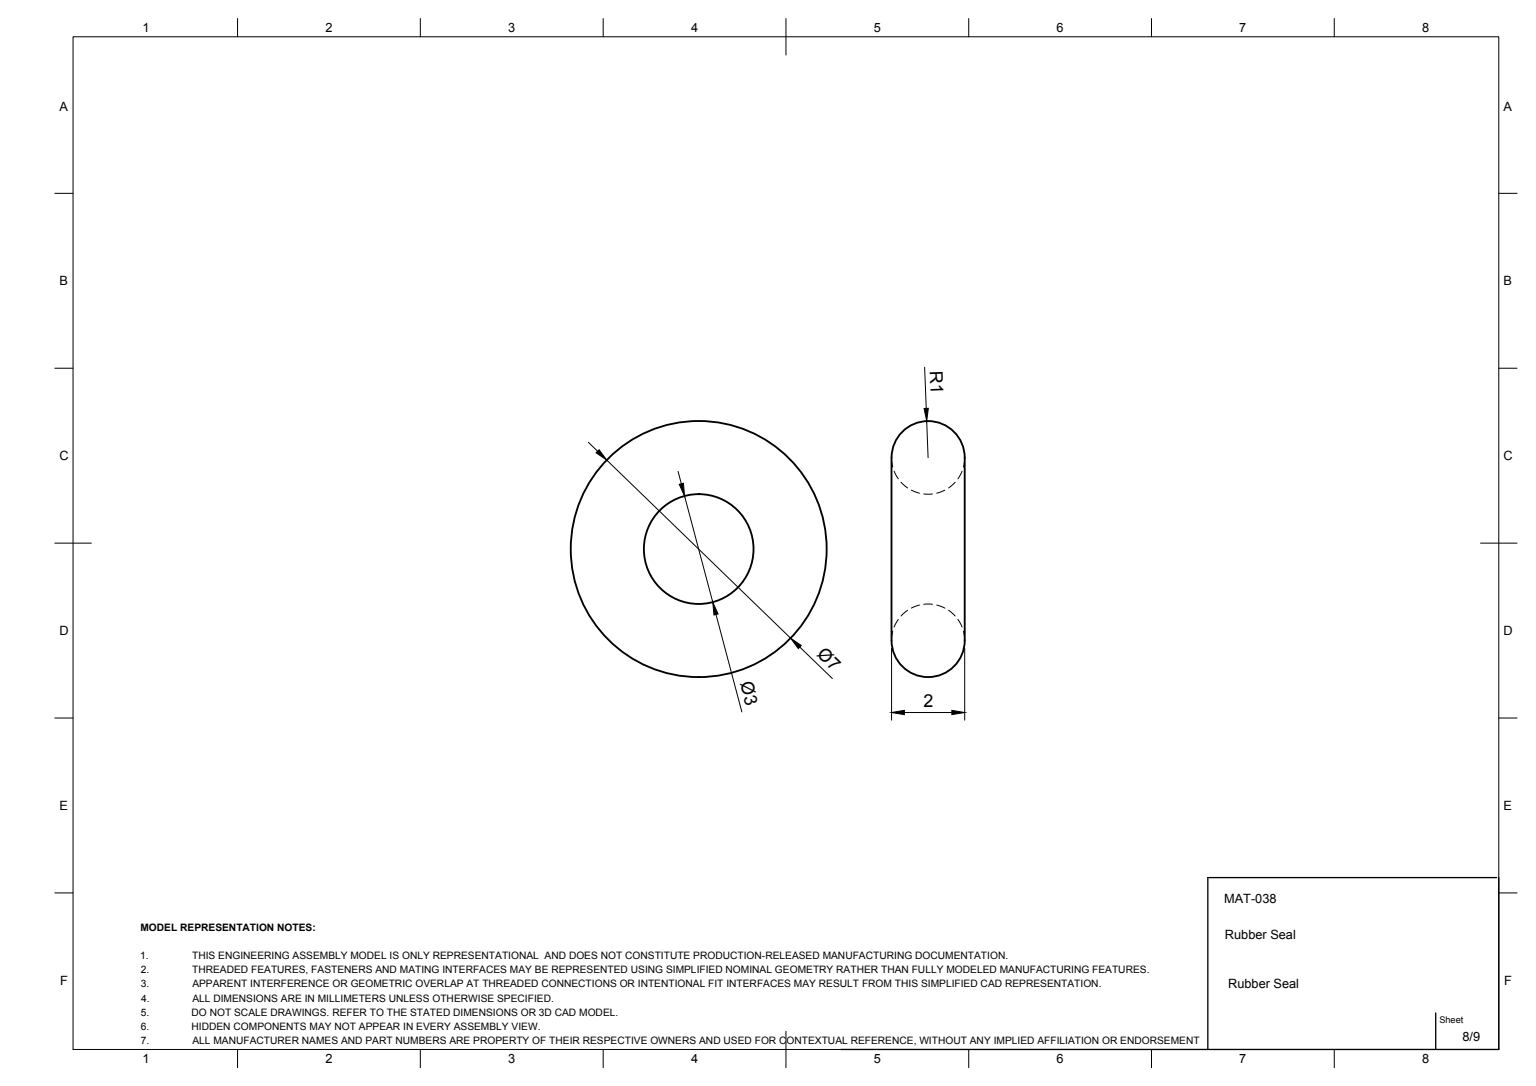
ISO-10303-21;
HEADER;
/* Generated by software containing ST-Developer
 * from STEP Tools, Inc. (www.steptools.com) 
 */

FILE_DESCRIPTION(
/* description */ ('STEP AP214'),
/* implementation_level */ '2;1');

FILE_NAME(
/* name */ 'Rubber Seal.step',
/* time_stamp */ '2026-11-14T21:32:33-08:00',
/* author */ (''),
/* organization */ (''),
/* preprocessor_version */ 'ST-DEVELOPER v20.2',
/* originating_system */ 'Autodesk Translation Framework v15.17.0.0',
/* authorisation */ '');

FILE_SCHEMA (('AUTOMOTIVE_DESIGN { 1 0 10303 214 3 1 1 }'));
ENDSEC;

DATA;
#10=MECHANICAL_DESIGN_GEOMETRIC_PRESENTATION_REPRESENTATION('',(#184),#10551);
#132=TOROIDAL_SURFACE('',#4013,2.5,1.);
#166=SHAPE_REPRESENTATION_RELATIONSHIP('SRR','None',#10593,#175);
#175=ADVANCED_BREP_SHAPE_REPRESENTATION('',(#194),#10549);
#184=STYLED_ITEM('',(#10644),#194);
#194=MANIFOLD_SOLID_BREP('Body1',#3433);
#508=FACE_OUTER_BOUND('',#754,.T.);
#754=EDGE_LOOP('',(#3122,#3123,#3124,#3125));
#1413=CIRCLE('',#4014,1.);
#1414=CIRCLE('',#4015,1.5);
#1698=VERTEX_POINT('',#8365);
#2174=EDGE_CURVE('',#1698,#1698,#1413,.T.);
#2175=EDGE_CURVE('',#1698,#1698,#1414,.T.);
#3122=ORIENTED_EDGE('',*,*,#2174,.F.);
#3123=ORIENTED_EDGE('',*,*,#2175,.T.);
#3124=ORIENTED_EDGE('',*,*,#2174,.T.);
#3125=ORIENTED_EDGE('',*,*,#2175,.F.);
#3420=ADVANCED_FACE('',(#508),#132,.T.);
#3433=CLOSED_SHELL('',(#3420));
#4012=AXIS2_PLACEMENT_3D('',#8363,#5185,#5186);
#4013=AXIS2_PLACEMENT_3D('',#8364,#5187,#5188);
#4014=AXIS2_PLACEMENT_3D('',#8366,#5189,#5190);
#4015=AXIS2_PLACEMENT_3D('',#8367,#5191,#5192);
#5185=DIRECTION('axis',(0.,0.,1.));
#5186=DIRECTION('refdir',(1.,0.,0.));
#5187=DIRECTION('center_axis',(0.,-1.,0.));
#5188=DIRECTION('ref_axis',(0.,0.,-1.));
#5189=DIRECTION('center_axis',(-1.,0.,-1.22464679914735E-16));
#5190=DIRECTION('ref_axis',(-1.22464679914735E-16,0.,1.));
#5191=DIRECTION('center_axis',(0.,1.,0.));
#5192=DIRECTION('ref_axis',(0.,0.,-1.));
#8363=CARTESIAN_POINT('',(0.,0.,0.));
#8364=CARTESIAN_POINT('Origin',(0.,0.,0.));
#8365=CARTESIAN_POINT('',(-1.83697019872103E-16,-1.22464679914735E-16,1.5));
#8366=CARTESIAN_POINT('Origin',(-3.06161699786838E-16,0.,2.5));
#8367=CARTESIAN_POINT('Origin',(0.,1.22464679914735E-16,0.));
#10538=UNCERTAINTY_MEASURE_WITH_UNIT(LENGTH_MEASURE(0.01),#10552,
'DISTANCE_ACCURACY_VALUE',
'Maximum model space distance between geometric entities at asserted c
onnectivities');
#10540=UNCERTAINTY_MEASURE_WITH_UNIT(LENGTH_MEASURE(0.01),#10552,
'DISTANCE_ACCURACY_VALUE',
'Maximum model space distance between geometric entities at asserted c
onnectivities');
#10549=(
GEOMETRIC_REPRESENTATION_CONTEXT(3)
GLOBAL_UNCERTAINTY_ASSIGNED_CONTEXT((#10538))
GLOBAL_UNIT_ASSIGNED_CONTEXT((#10552,#10554,#10555))
REPRESENTATION_CONTEXT('','3D')
);
#10551=(
GEOMETRIC_REPRESENTATION_CONTEXT(3)
GLOBAL_UNCERTAINTY_ASSIGNED_CONTEXT((#10540))
GLOBAL_UNIT_ASSIGNED_CONTEXT((#10552,#10554,#10555))
REPRESENTATION_CONTEXT('','3D')
);
#10552=(
LENGTH_UNIT()
NAMED_UNIT(*)
SI_UNIT(.MILLI.,.METRE.)
);
#10554=(
NAMED_UNIT(*)
PLANE_ANGLE_UNIT()
SI_UNIT($,.RADIAN.)
);
#10555=(
NAMED_UNIT(*)
SI_UNIT($,.STERADIAN.)
SOLID_ANGLE_UNIT()
);
#10564=SHAPE_DEFINITION_REPRESENTATION(#10574,#10593);
#10574=PRODUCT_DEFINITION_SHAPE('',$,#10604);
#10593=SHAPE_REPRESENTATION('',(#4012),#10549);
#10595=PRODUCT_DEFINITION_CONTEXT('part definition',#10627,'design');
#10604=PRODUCT_DEFINITION('Rubber Seal','Rubber Seal',#10614,#10595);
#10614=PRODUCT_DEFINITION_FORMATION('',$,#10637);
#10627=APPLICATION_CONTEXT(
'Core Data for Automotive Mechanical Design Process');
#10628=PRODUCT_CONTEXT('part definition',#10627,'mechanical');
#10637=PRODUCT('Rubber Seal','Rubber Seal',$,(#10628));
#10644=PRESENTATION_STYLE_ASSIGNMENT((#10651));
#10651=SURFACE_STYLE_USAGE(.BOTH.,#10658);
#10658=SURFACE_SIDE_STYLE('',(#10665));
#10665=SURFACE_STYLE_FILL_AREA(#10672);
#10672=FILL_AREA_STYLE('Opaque(31,36,43)',(#10679));
#10679=FILL_AREA_STYLE_COLOUR('Opaque(31,36,43)',#10686);
#10686=COLOUR_RGB('Opaque(31,36,43)',0.12156862745098,0.141176470588235,
0.168627450980392);
ENDSEC;
END-ISO-10303-21;
